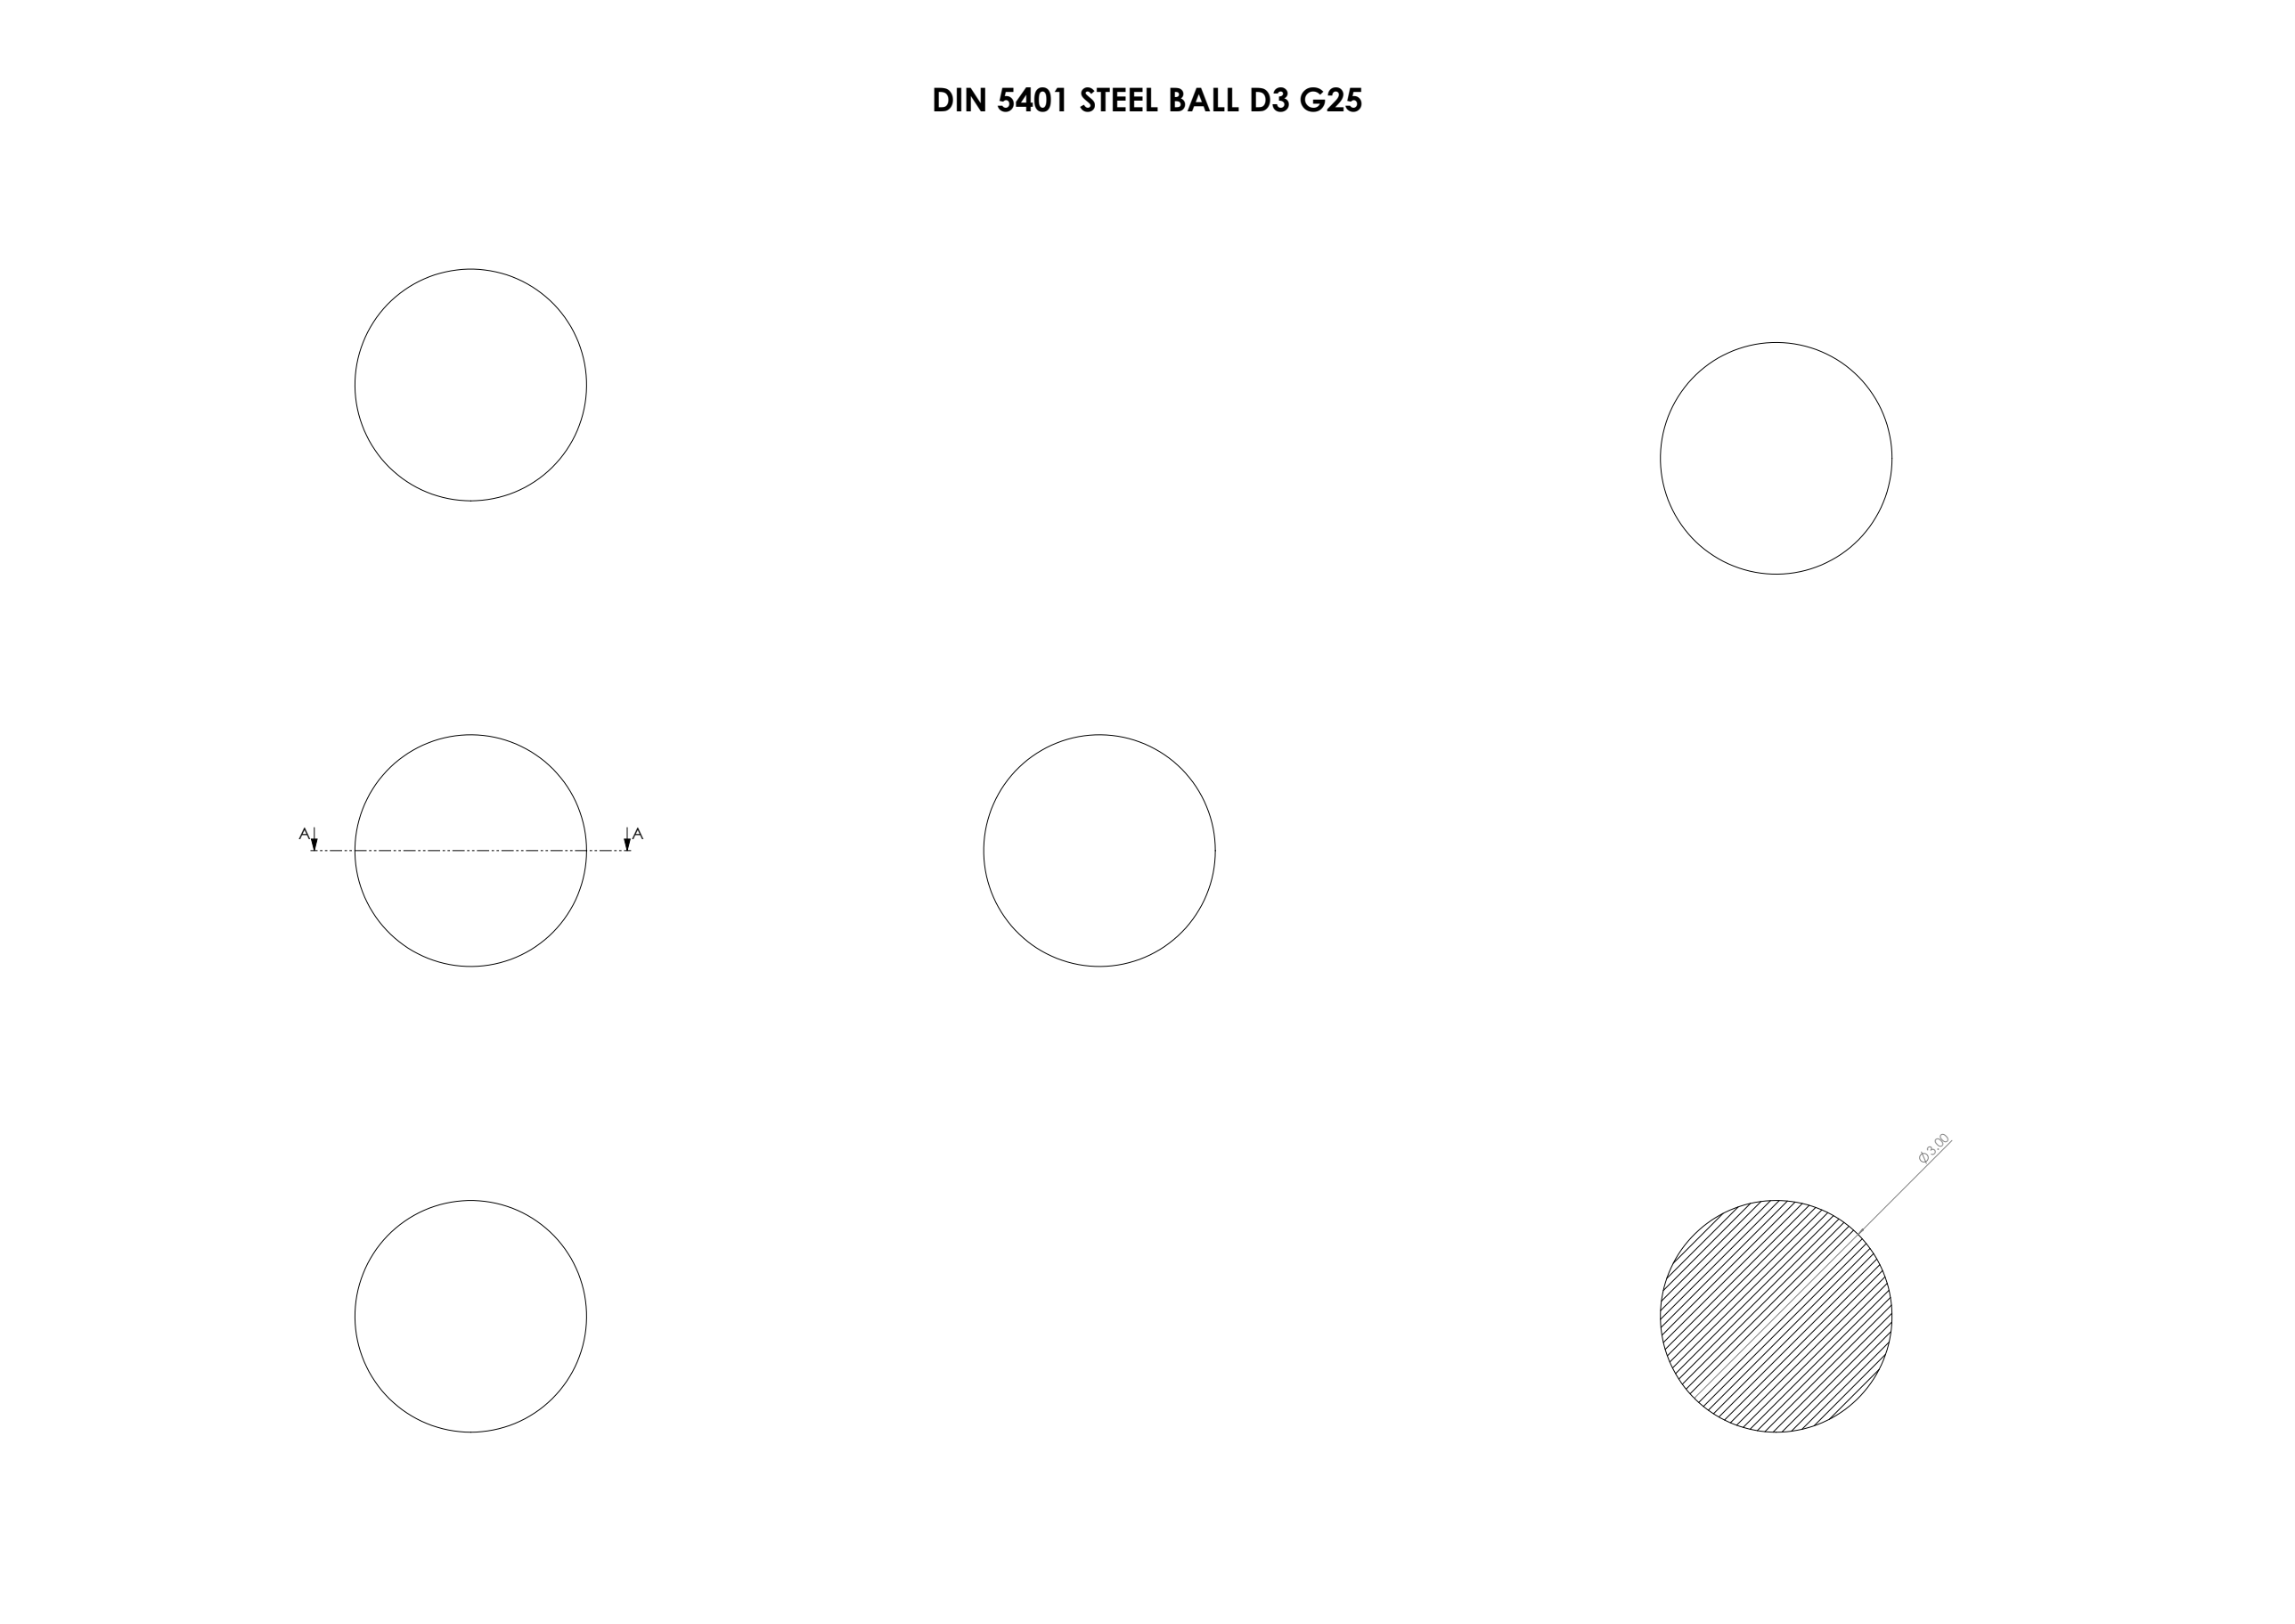
ISO-10303-21;
HEADER;
/* Generated by software containing ST-Developer
 * from STEP Tools, Inc. (www.steptools.com) 
 */

FILE_DESCRIPTION(
/* description */ (''),
/* implementation_level */ '2;1');

FILE_NAME(
/* name */ 
'09_DIN_5401_Steel_Ball_D3_G25.step',
/* time_stamp */ '2026-10-20T10:06:23-07:00',
/* author */ (''),
/* organization */ (''),
/* preprocessor_version */ 'ST-DEVELOPER v20.2',
/* originating_system */ 'Autodesk Translation Framework v15.15.0.0',
/* authorisation */ '');

FILE_SCHEMA (('AUTOMOTIVE_DESIGN { 1 0 10303 214 3 1 1 }'));
ENDSEC;

DATA;
#10=MECHANICAL_DESIGN_GEOMETRIC_PRESENTATION_REPRESENTATION('',(#470),#38611);
#95=SPHERICAL_SURFACE('',#17325,0.15);
#442=SHAPE_REPRESENTATION_RELATIONSHIP('SRR','None',#38678,#456);
#456=ADVANCED_BREP_SHAPE_REPRESENTATION('',(#484),#38607);
#470=STYLED_ITEM('',(#38864),#484);
#484=MANIFOLD_SOLID_BREP('Ball',#16244);
#1515=CIRCLE('',#17326,0.15);
#2387=FACE_OUTER_BOUND('',#3347,.T.);
#3347=EDGE_LOOP('',(#13115,#13116));
#7072=VERTEX_POINT('',#31610);
#7073=VERTEX_POINT('',#31611);
#9173=EDGE_CURVE('',#7072,#7073,#1515,.T.);
#13115=ORIENTED_EDGE('',*,*,#9173,.T.);
#13116=ORIENTED_EDGE('',*,*,#9173,.F.);
#15930=ADVANCED_FACE('',(#2387),#95,.T.);
#16244=CLOSED_SHELL('',(#15930));
#17324=AXIS2_PLACEMENT_3D('',#31608,#20511,#20512);
#17325=AXIS2_PLACEMENT_3D('',#31609,#20513,#20514);
#17326=AXIS2_PLACEMENT_3D('',#31612,#20515,#20516);
#20511=DIRECTION('axis',(0.,0.,1.));
#20512=DIRECTION('refdir',(1.,0.,0.));
#20513=DIRECTION('center_axis',(6.12323399573677E-17,0.,1.));
#20514=DIRECTION('ref_axis',(1.,0.,0.));
#20515=DIRECTION('center_axis',(1.22464679914735E-16,-1.,0.));
#20516=DIRECTION('ref_axis',(-1.,-1.22464679914735E-16,0.));
#31608=CARTESIAN_POINT('',(0.,0.,0.));
#31609=CARTESIAN_POINT('Origin',(0.,0.,0.));
#31610=CARTESIAN_POINT('',(-9.18485099360515E-18,-1.12481983699639E-33,
0.15));
#31611=CARTESIAN_POINT('',(-9.18485099360515E-18,-1.12481983699639E-33,
-0.15));
#31612=CARTESIAN_POINT('Origin',(0.,0.,0.));
#38591=UNCERTAINTY_MEASURE_WITH_UNIT(LENGTH_MEASURE(0.001),#38612,
'DISTANCE_ACCURACY_VALUE',
'Maximum model space distance between geometric entities at asserted c
onnectivities');
#38595=UNCERTAINTY_MEASURE_WITH_UNIT(LENGTH_MEASURE(0.001),#38612,
'DISTANCE_ACCURACY_VALUE',
'Maximum model space distance between geometric entities at asserted c
onnectivities');
#38607=(
GEOMETRIC_REPRESENTATION_CONTEXT(3)
GLOBAL_UNCERTAINTY_ASSIGNED_CONTEXT((#38591))
GLOBAL_UNIT_ASSIGNED_CONTEXT((#38612,#38614,#38615))
REPRESENTATION_CONTEXT('','3D')
);
#38611=(
GEOMETRIC_REPRESENTATION_CONTEXT(3)
GLOBAL_UNCERTAINTY_ASSIGNED_CONTEXT((#38595))
GLOBAL_UNIT_ASSIGNED_CONTEXT((#38612,#38614,#38615))
REPRESENTATION_CONTEXT('','3D')
);
#38612=(
LENGTH_UNIT()
NAMED_UNIT(*)
SI_UNIT(.CENTI.,.METRE.)
);
#38614=(
NAMED_UNIT(*)
PLANE_ANGLE_UNIT()
SI_UNIT($,.RADIAN.)
);
#38615=(
NAMED_UNIT(*)
SI_UNIT($,.STERADIAN.)
SOLID_ANGLE_UNIT()
);
#38627=SHAPE_DEFINITION_REPRESENTATION(#38642,#38678);
#38642=PRODUCT_DEFINITION_SHAPE('',$,#38694);
#38678=SHAPE_REPRESENTATION('',(#17324),#38607);
#38682=PRODUCT_DEFINITION_CONTEXT('part definition',#38729,'design');
#38694=PRODUCT_DEFINITION('2026-10-19-02-31-51-310',
'09_DIN_5401_Steel_Ball_D3_G25',#38709,#38682);
#38709=PRODUCT_DEFINITION_FORMATION('',$,#38742);
#38729=APPLICATION_CONTEXT(
'Core Data for Automotive Mechanical Design Process');
#38730=PRODUCT_CONTEXT('part definition',#38729,'mechanical');
#38742=PRODUCT('2026-10-19-02-31-51-310',
'09_DIN_5401_Steel_Ball_D3_G25',$,(#38730));
#38858=COLOUR_RGB('Light Blue',0.38,0.62,0.78);
#38859=FILL_AREA_STYLE_COLOUR('',#38858);
#38860=FILL_AREA_STYLE('',(#38859));
#38861=SURFACE_STYLE_FILL_AREA(#38860);
#38862=SURFACE_SIDE_STYLE('',(#38861));
#38863=SURFACE_STYLE_USAGE(.BOTH.,#38862);
#38864=PRESENTATION_STYLE_ASSIGNMENT((#38863));
ENDSEC;
END-ISO-10303-21;
